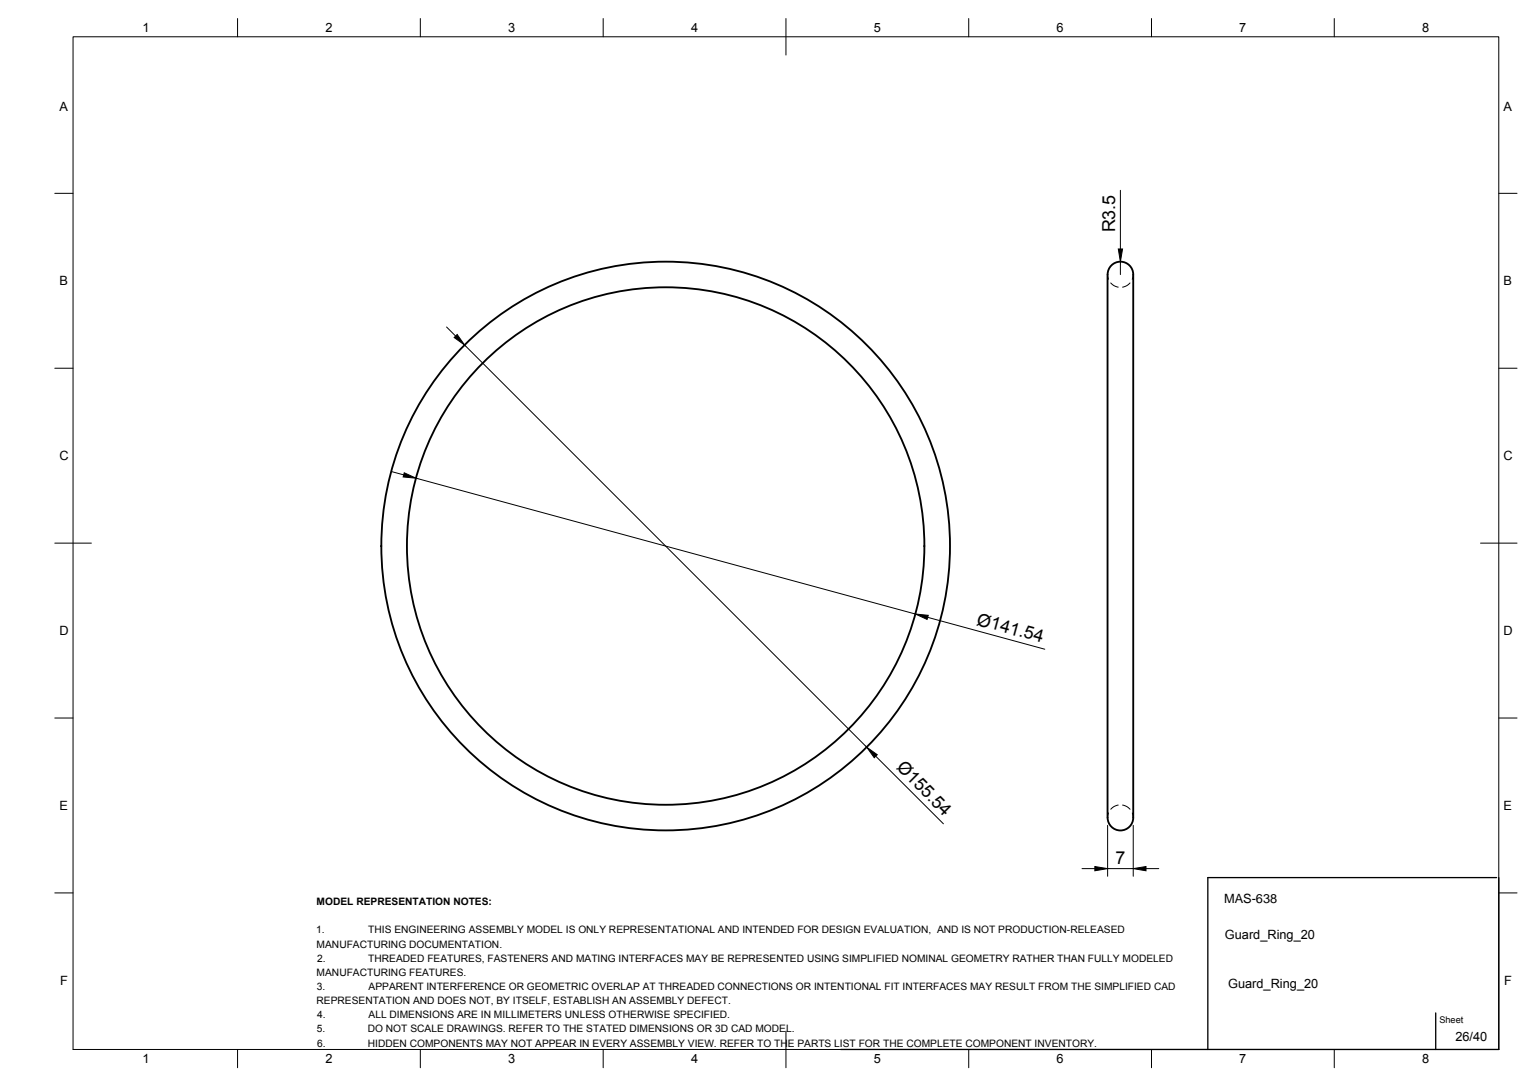
ISO-10303-21;
HEADER;
FILE_DESCRIPTION((''),'2;1');
FILE_NAME('Guard_Ring_20.step','2026-10-09T12:00:21-07:00',(''),(''),'','','');
FILE_SCHEMA (('AUTOMOTIVE_DESIGN { 1 0 10303 214 3 1 1 }'));
ENDSEC;
DATA;
#10=MECHANICAL_DESIGN_GEOMETRIC_PRESENTATION_REPRESENTATION('',(#425),#10334);
#353=SHAPE_REPRESENTATION_RELATIONSHIP('SRR','None',#10469,#385) ;
#385=ADVANCED_BREP_SHAPE_REPRESENTATION('',(#457),#10321) ;
#425=STYLED_ITEM('',(#10631),#457) ;
#457=MANIFOLD_SOLID_BREP('Body1',#3579) ;
#878=FACE_OUTER_BOUND('',#1078,.T.) ;
#1078=EDGE_LOOP('',(#2425,#2426,#2427,#2428)) ;
#1314=CIRCLE('',#4051,0.349999999999999) ;
#1315=CIRCLE('',#4052,7.07681446136678) ;
#1532=VERTEX_POINT('',#5748) ;
#1869=EDGE_CURVE('',#1532,#1532,#1314,.T.) ;
#1870=EDGE_CURVE('',#1532,#1532,#1315,.T.) ;
#2425=ORIENTED_EDGE('',*,*,#1869,.F.) ;
#2426=ORIENTED_EDGE('',*,*,#1870,.T.) ;
#2427=ORIENTED_EDGE('',*,*,#1869,.T.) ;
#2428=ORIENTED_EDGE('',*,*,#1870,.F.) ;
#3324=TOROIDAL_SURFACE('',#4050,7.42681446136678,0.349999999999999) ;
#3386=ADVANCED_FACE('',(#878),#3324,.T.) ;
#3579=CLOSED_SHELL('',(#3386)) ;
#4049=AXIS2_PLACEMENT_3D('',#5746,#4659,#4660) ;
#4050=AXIS2_PLACEMENT_3D('',#5747,#4661,#4662) ;
#4051=AXIS2_PLACEMENT_3D('',#5749,#4663,#4664) ;
#4052=AXIS2_PLACEMENT_3D('',#5750,#4665,#4666) ;
#4659=DIRECTION('axis',(0.,0.,1.)) ;
#4660=DIRECTION('refdir',(1.,0.,0.)) ;
#4661=DIRECTION('center_axis',(-6.42891162084177E-17,-1.,-1.01883556321148E-16)) ;
#4662=DIRECTION('ref_axis',(1.,0.,0.)) ;
#4663=DIRECTION('center_axis',(0.,1.01883556321148E-16,-1.)) ;
#4664=DIRECTION('ref_axis',(-1.,0.,0.)) ;
#4665=DIRECTION('center_axis',(6.42891162084177E-17,1.,1.01883556321148E-16)) ;
#4666=DIRECTION('ref_axis',(1.,-6.42891162084177E-17,-6.55000379205715E-33)) ;
#5746=CARTESIAN_POINT('',(0.,0.,0.)) ;
#5747=CARTESIAN_POINT('Origin',(23.47768801576,63.8831179463143,68.2224337400009)) ;
#5748=CARTESIAN_POINT('',(16.4008735543932,63.8831179463143,68.2224337400009)) ;
#5749=CARTESIAN_POINT('Origin',(16.0508735543932,63.8831179463143,68.2224337400009)) ;
#5750=CARTESIAN_POINT('Origin',(23.47768801576,63.8831179463143,68.2224337400009)) ;
#10284=UNCERTAINTY_MEASURE_WITH_UNIT(LENGTH_MEASURE(0.001),#10335,
'DISTANCE_ACCURACY_VALUE',
'Maximum model space distance between geometric entities at asserted c
onnectivities') ;
#10297=UNCERTAINTY_MEASURE_WITH_UNIT(LENGTH_MEASURE(0.001),#10335,
'DISTANCE_ACCURACY_VALUE',
'Maximum model space distance between geometric entities at asserted c
onnectivities') ;
#10321=(
GEOMETRIC_REPRESENTATION_CONTEXT(3)
GLOBAL_UNCERTAINTY_ASSIGNED_CONTEXT((#10284))
GLOBAL_UNIT_ASSIGNED_CONTEXT((#10335,#10337,#10338))
REPRESENTATION_CONTEXT('','3D')
) ;
#10334=(
GEOMETRIC_REPRESENTATION_CONTEXT(3)
GLOBAL_UNCERTAINTY_ASSIGNED_CONTEXT((#10297))
GLOBAL_UNIT_ASSIGNED_CONTEXT((#10335,#10337,#10338))
REPRESENTATION_CONTEXT('','3D')
) ;
#10335=(
LENGTH_UNIT()
NAMED_UNIT(*)
SI_UNIT(.CENTI.,.METRE.)
) ;
#10337=(
NAMED_UNIT(*)
PLANE_ANGLE_UNIT()
SI_UNIT($,.RADIAN.)
) ;
#10338=(
NAMED_UNIT(*)
SI_UNIT($,.STERADIAN.)
SOLID_ANGLE_UNIT()
) ;
#10362=SHAPE_DEFINITION_REPRESENTATION(#10398,#10469) ;
#10398=PRODUCT_DEFINITION_SHAPE('',$,#10506) ;
#10469=SHAPE_REPRESENTATION('',(#4049),#10321) ;
#10482=PRODUCT_DEFINITION_CONTEXT('part definition',#10592,'design') ;
#10506=PRODUCT_DEFINITION('Guard_Ring_20','Guard_Ring_20',#10542,#10482) ;
#10542=PRODUCT_DEFINITION_FORMATION('',$,#10617) ;
#10592=APPLICATION_CONTEXT(
'Core Data for Automotive Mechanical Design Process') ;
#10593=PRODUCT_CONTEXT('part definition',#10592,'mechanical') ;
#10617=PRODUCT('Guard_Ring_20','Guard_Ring_20',$,(#10593)) ;
#10631=PRESENTATION_STYLE_ASSIGNMENT((#10635)) ;
#10635=SURFACE_STYLE_USAGE(.BOTH.,#10639) ;
#10639=SURFACE_SIDE_STYLE('',(#10643)) ;
#10643=SURFACE_STYLE_FILL_AREA(#10647) ;
#10647=FILL_AREA_STYLE('Opaque(25,25,25)',(#10651)) ;
#10651=FILL_AREA_STYLE_COLOUR('Opaque(25,25,25)',#10655) ;
#10655=COLOUR_RGB('Opaque(25,25,25)', 0.09019608, 0.27058824, 0.51372549) ;
ENDSEC;
END-ISO-10303-21;
